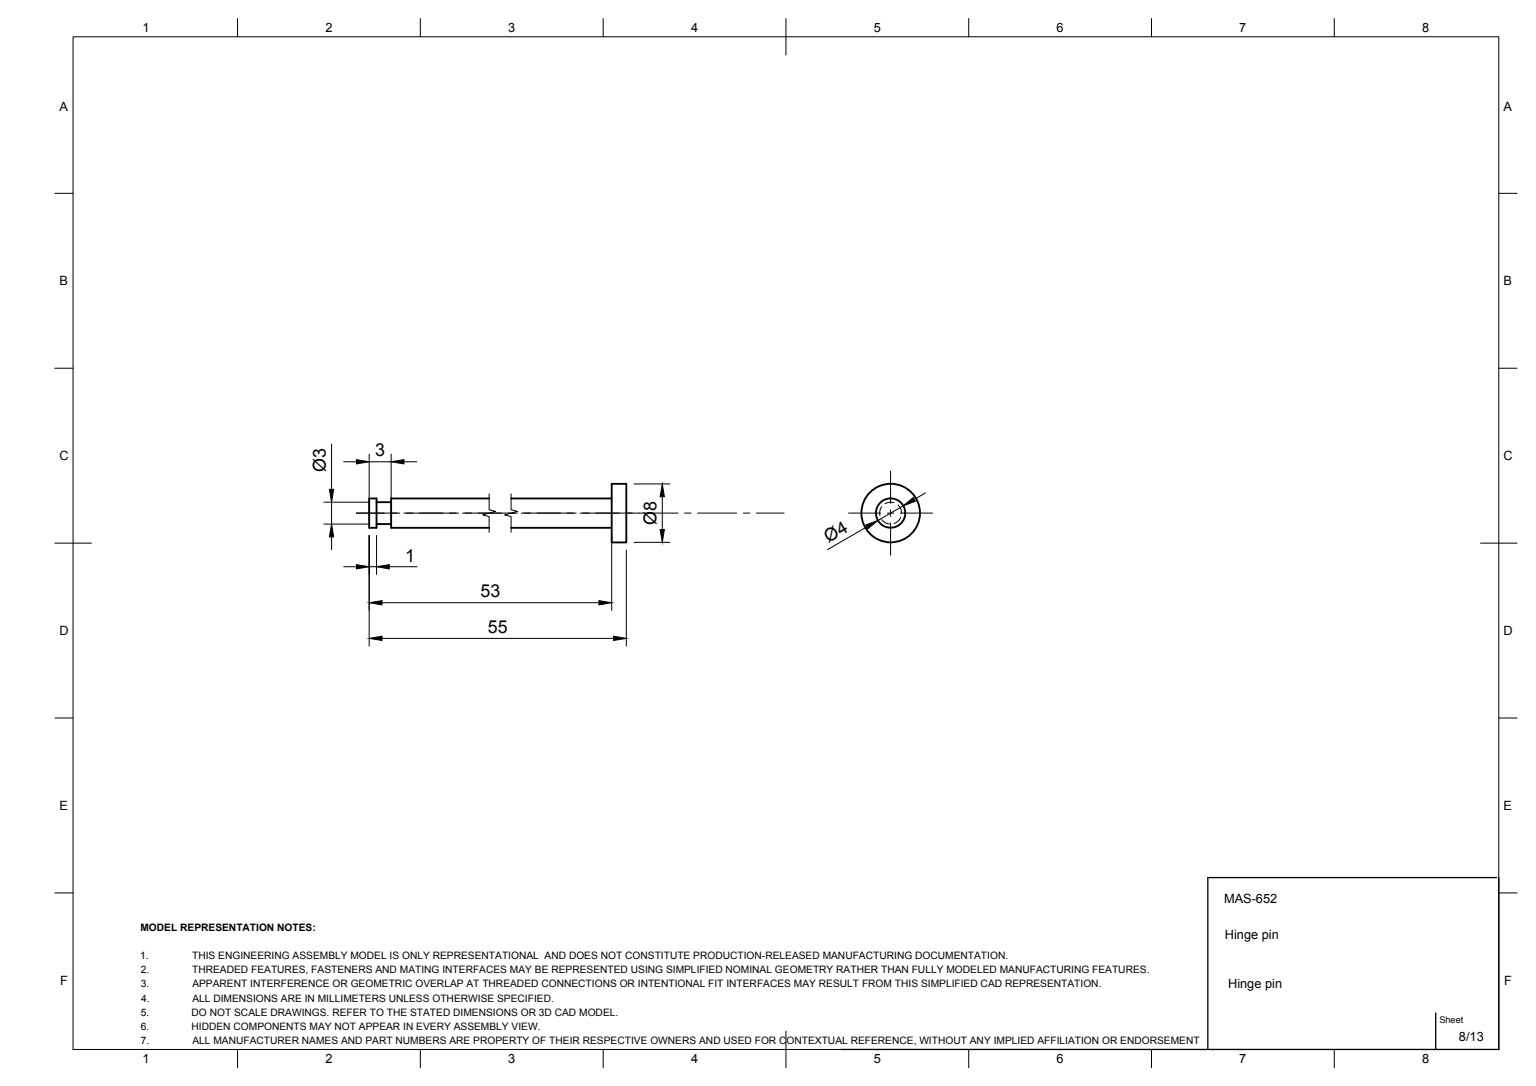
ISO-10303-21;
HEADER;
/* Generated by software containing ST-Developer
 * from STEP Tools, Inc. (www.steptools.com) 
 */

FILE_DESCRIPTION(
/* description */ ('Independent hinged machine back cover with retained hinge pins, perim
eter gasket and quarter-turn cam latch. Nominal cover 360 x 260 x 3 mm
, frame 430 x 300 x 20 mm. No guarding, structural or ingress rating a
ssigned.'),
/* implementation_level */ '2;1');

FILE_NAME(
/* name */ 'Hinge pin.step',
/* time_stamp */ '2026-11-09T19:36:59-08:00',
/* author */ (''),
/* organization */ (''),
/* preprocessor_version */ 'ST-DEVELOPER v20.2',
/* originating_system */ 'Autodesk Translation Framework v15.17.0.0',
/* authorisation */ '');

FILE_SCHEMA (('AUTOMOTIVE_DESIGN { 1 0 10303 214 3 1 1 }'));
ENDSEC;

DATA;
#10=MECHANICAL_DESIGN_GEOMETRIC_PRESENTATION_REPRESENTATION('',(#208),#32627);
#172=SHAPE_REPRESENTATION_RELATIONSHIP('SRR','None',#32718,#190);
#190=ADVANCED_BREP_SHAPE_REPRESENTATION('',(#226),#32619);
#208=STYLED_ITEM('',(#32812),#226);
#226=MANIFOLD_SOLID_BREP('Body1',#8685);
#274=FACE_BOUND('',#1294,.T.);
#275=FACE_BOUND('',#1296,.T.);
#276=FACE_BOUND('',#1299,.T.);
#402=PLANE('',#9298);
#403=PLANE('',#9300);
#404=PLANE('',#9304);
#405=PLANE('',#9309);
#406=PLANE('',#9311);
#777=FACE_OUTER_BOUND('',#1292,.T.);
#778=FACE_OUTER_BOUND('',#1293,.T.);
#779=FACE_OUTER_BOUND('',#1295,.T.);
#780=FACE_OUTER_BOUND('',#1297,.T.);
#781=FACE_OUTER_BOUND('',#1298,.T.);
#782=FACE_OUTER_BOUND('',#1300,.T.);
#783=FACE_OUTER_BOUND('',#1301,.T.);
#784=FACE_OUTER_BOUND('',#1302,.T.);
#785=FACE_OUTER_BOUND('',#1303,.T.);
#1292=EDGE_LOOP('',(#7125,#7126,#7127,#7128));
#1293=EDGE_LOOP('',(#7129));
#1294=EDGE_LOOP('',(#7130));
#1295=EDGE_LOOP('',(#7131));
#1296=EDGE_LOOP('',(#7132));
#1297=EDGE_LOOP('',(#7133,#7134,#7135,#7136));
#1298=EDGE_LOOP('',(#7137));
#1299=EDGE_LOOP('',(#7138));
#1300=EDGE_LOOP('',(#7139,#7140,#7141,#7142));
#1301=EDGE_LOOP('',(#7143));
#1302=EDGE_LOOP('',(#7144,#7145,#7146,#7147));
#1303=EDGE_LOOP('',(#7148));
#1539=CIRCLE('',#9296,1.5);
#1540=CIRCLE('',#9297,1.5);
#1541=CIRCLE('',#9299,2.);
#1542=CIRCLE('',#9301,2.);
#1543=CIRCLE('',#9303,2.);
#1544=CIRCLE('',#9305,4.);
#1545=CIRCLE('',#9306,2.);
#1546=CIRCLE('',#9308,4.);
#2552=LINE('',#26260,#3098);
#2553=LINE('',#26271,#3099);
#2554=LINE('',#26279,#3100);
#2555=LINE('',#26283,#3101);
#3098=VECTOR('',#10716,1.5);
#3099=VECTOR('',#10731,2.);
#3100=VECTOR('',#10740,4.);
#3101=VECTOR('',#10747,2.);
#3853=VERTEX_POINT('',#26257);
#3854=VERTEX_POINT('',#26259);
#3855=VERTEX_POINT('',#26263);
#3856=VERTEX_POINT('',#26266);
#3857=VERTEX_POINT('',#26269);
#3858=VERTEX_POINT('',#26273);
#3859=VERTEX_POINT('',#26275);
#3860=VERTEX_POINT('',#26278);
#4986=EDGE_CURVE('',#3853,#3853,#1539,.T.);
#4987=EDGE_CURVE('',#3853,#3854,#2552,.T.);
#4988=EDGE_CURVE('',#3854,#3854,#1540,.T.);
#4989=EDGE_CURVE('',#3855,#3855,#1541,.T.);
#4990=EDGE_CURVE('',#3856,#3856,#1542,.T.);
#4991=EDGE_CURVE('',#3857,#3857,#1543,.T.);
#4992=EDGE_CURVE('',#3857,#3856,#2553,.T.);
#4993=EDGE_CURVE('',#3858,#3858,#1544,.T.);
#4994=EDGE_CURVE('',#3859,#3859,#1545,.T.);
#4995=EDGE_CURVE('',#3858,#3860,#2554,.T.);
#4996=EDGE_CURVE('',#3860,#3860,#1546,.T.);
#4997=EDGE_CURVE('',#3855,#3859,#2555,.T.);
#7125=ORIENTED_EDGE('',*,*,#4986,.T.);
#7126=ORIENTED_EDGE('',*,*,#4987,.T.);
#7127=ORIENTED_EDGE('',*,*,#4988,.F.);
#7128=ORIENTED_EDGE('',*,*,#4987,.F.);
#7129=ORIENTED_EDGE('',*,*,#4989,.F.);
#7130=ORIENTED_EDGE('',*,*,#4986,.F.);
#7131=ORIENTED_EDGE('',*,*,#4990,.F.);
#7132=ORIENTED_EDGE('',*,*,#4988,.T.);
#7133=ORIENTED_EDGE('',*,*,#4991,.F.);
#7134=ORIENTED_EDGE('',*,*,#4992,.T.);
#7135=ORIENTED_EDGE('',*,*,#4990,.T.);
#7136=ORIENTED_EDGE('',*,*,#4992,.F.);
#7137=ORIENTED_EDGE('',*,*,#4993,.T.);
#7138=ORIENTED_EDGE('',*,*,#4994,.F.);
#7139=ORIENTED_EDGE('',*,*,#4993,.F.);
#7140=ORIENTED_EDGE('',*,*,#4995,.T.);
#7141=ORIENTED_EDGE('',*,*,#4996,.T.);
#7142=ORIENTED_EDGE('',*,*,#4995,.F.);
#7143=ORIENTED_EDGE('',*,*,#4996,.F.);
#7144=ORIENTED_EDGE('',*,*,#4989,.T.);
#7145=ORIENTED_EDGE('',*,*,#4997,.T.);
#7146=ORIENTED_EDGE('',*,*,#4994,.T.);
#7147=ORIENTED_EDGE('',*,*,#4997,.F.);
#7148=ORIENTED_EDGE('',*,*,#4991,.T.);
#8108=CYLINDRICAL_SURFACE('',#9295,1.5);
#8109=CYLINDRICAL_SURFACE('',#9302,2.);
#8110=CYLINDRICAL_SURFACE('',#9307,4.);
#8111=CYLINDRICAL_SURFACE('',#9310,2.);
#8525=ADVANCED_FACE('',(#777),#8108,.T.);
#8526=ADVANCED_FACE('',(#778,#274),#402,.F.);
#8527=ADVANCED_FACE('',(#779,#275),#403,.F.);
#8528=ADVANCED_FACE('',(#780),#8109,.T.);
#8529=ADVANCED_FACE('',(#781,#276),#404,.T.);
#8530=ADVANCED_FACE('',(#782),#8110,.T.);
#8531=ADVANCED_FACE('',(#783),#405,.F.);
#8532=ADVANCED_FACE('',(#784),#8111,.T.);
#8533=ADVANCED_FACE('',(#785),#406,.T.);
#8685=CLOSED_SHELL('',(#8525,#8526,#8527,#8528,#8529,#8530,#8531,#8532,
#8533));
#9294=AXIS2_PLACEMENT_3D('',#26255,#10710,#10711);
#9295=AXIS2_PLACEMENT_3D('',#26256,#10712,#10713);
#9296=AXIS2_PLACEMENT_3D('',#26258,#10714,#10715);
#9297=AXIS2_PLACEMENT_3D('',#26261,#10717,#10718);
#9298=AXIS2_PLACEMENT_3D('',#26262,#10719,#10720);
#9299=AXIS2_PLACEMENT_3D('',#26264,#10721,#10722);
#9300=AXIS2_PLACEMENT_3D('',#26265,#10723,#10724);
#9301=AXIS2_PLACEMENT_3D('',#26267,#10725,#10726);
#9302=AXIS2_PLACEMENT_3D('',#26268,#10727,#10728);
#9303=AXIS2_PLACEMENT_3D('',#26270,#10729,#10730);
#9304=AXIS2_PLACEMENT_3D('',#26272,#10732,#10733);
#9305=AXIS2_PLACEMENT_3D('',#26274,#10734,#10735);
#9306=AXIS2_PLACEMENT_3D('',#26276,#10736,#10737);
#9307=AXIS2_PLACEMENT_3D('',#26277,#10738,#10739);
#9308=AXIS2_PLACEMENT_3D('',#26280,#10741,#10742);
#9309=AXIS2_PLACEMENT_3D('',#26281,#10743,#10744);
#9310=AXIS2_PLACEMENT_3D('',#26282,#10745,#10746);
#9311=AXIS2_PLACEMENT_3D('',#26284,#10748,#10749);
#10710=DIRECTION('axis',(0.,0.,1.));
#10711=DIRECTION('refdir',(1.,0.,0.));
#10712=DIRECTION('center_axis',(0.,0.,1.));
#10713=DIRECTION('ref_axis',(1.,0.,0.));
#10714=DIRECTION('center_axis',(0.,0.,1.));
#10715=DIRECTION('ref_axis',(1.,0.,0.));
#10716=DIRECTION('',(0.,0.,1.));
#10717=DIRECTION('center_axis',(0.,0.,1.));
#10718=DIRECTION('ref_axis',(1.,0.,0.));
#10719=DIRECTION('center_axis',(0.,0.,-1.));
#10720=DIRECTION('ref_axis',(-1.,0.,0.));
#10721=DIRECTION('center_axis',(0.,0.,-1.));
#10722=DIRECTION('ref_axis',(1.,0.,0.));
#10723=DIRECTION('center_axis',(0.,0.,1.));
#10724=DIRECTION('ref_axis',(1.,0.,0.));
#10725=DIRECTION('center_axis',(0.,0.,1.));
#10726=DIRECTION('ref_axis',(1.,0.,0.));
#10727=DIRECTION('center_axis',(0.,0.,1.));
#10728=DIRECTION('ref_axis',(1.,0.,0.));
#10729=DIRECTION('center_axis',(0.,0.,1.));
#10730=DIRECTION('ref_axis',(1.,0.,0.));
#10731=DIRECTION('',(0.,0.,-1.));
#10732=DIRECTION('center_axis',(0.,0.,1.));
#10733=DIRECTION('ref_axis',(1.,0.,0.));
#10734=DIRECTION('center_axis',(0.,0.,1.));
#10735=DIRECTION('ref_axis',(1.,0.,0.));
#10736=DIRECTION('center_axis',(0.,0.,1.));
#10737=DIRECTION('ref_axis',(1.,0.,0.));
#10738=DIRECTION('center_axis',(0.,0.,1.));
#10739=DIRECTION('ref_axis',(1.,0.,0.));
#10740=DIRECTION('',(0.,0.,-1.));
#10741=DIRECTION('center_axis',(0.,0.,1.));
#10742=DIRECTION('ref_axis',(1.,0.,0.));
#10743=DIRECTION('center_axis',(0.,0.,1.));
#10744=DIRECTION('ref_axis',(1.,0.,0.));
#10745=DIRECTION('center_axis',(0.,0.,1.));
#10746=DIRECTION('ref_axis',(1.,0.,0.));
#10747=DIRECTION('',(0.,0.,-1.));
#10748=DIRECTION('center_axis',(0.,0.,1.));
#10749=DIRECTION('ref_axis',(1.,0.,0.));
#26255=CARTESIAN_POINT('',(0.,0.,0.));
#26256=CARTESIAN_POINT('Origin',(0.,0.,51.));
#26257=CARTESIAN_POINT('',(-1.5,-1.83697019872103E-16,50.));
#26258=CARTESIAN_POINT('Origin',(0.,0.,50.));
#26259=CARTESIAN_POINT('',(-1.5,-1.83697019872103E-16,52.));
#26260=CARTESIAN_POINT('',(-1.5,-1.83697019872103E-16,51.));
#26261=CARTESIAN_POINT('Origin',(0.,0.,52.));
#26262=CARTESIAN_POINT('Origin',(5.5,0.,50.));
#26263=CARTESIAN_POINT('',(-2.,2.44929359829471E-16,50.));
#26264=CARTESIAN_POINT('Origin',(0.,0.,50.));
#26265=CARTESIAN_POINT('Origin',(1.5,0.,52.));
#26266=CARTESIAN_POINT('',(-2.,-2.44929359829471E-16,52.));
#26267=CARTESIAN_POINT('Origin',(0.,0.,52.));
#26268=CARTESIAN_POINT('Origin',(0.,0.,0.));
#26269=CARTESIAN_POINT('',(-2.,-2.44929359829471E-16,53.));
#26270=CARTESIAN_POINT('Origin',(0.,0.,53.));
#26271=CARTESIAN_POINT('',(-2.,-2.44929359829471E-16,0.));
#26272=CARTESIAN_POINT('Origin',(0.,0.,0.));
#26273=CARTESIAN_POINT('',(-4.,-4.89858719658941E-16,0.));
#26274=CARTESIAN_POINT('Origin',(0.,0.,0.));
#26275=CARTESIAN_POINT('',(-2.,-2.44929359829471E-16,0.));
#26276=CARTESIAN_POINT('Origin',(0.,0.,0.));
#26277=CARTESIAN_POINT('Origin',(0.,0.,-2.));
#26278=CARTESIAN_POINT('',(-4.,-4.89858719658941E-16,-2.));
#26279=CARTESIAN_POINT('',(-4.,-4.89858719658941E-16,-2.));
#26280=CARTESIAN_POINT('Origin',(0.,0.,-2.));
#26281=CARTESIAN_POINT('Origin',(0.,0.,-2.));
#26282=CARTESIAN_POINT('Origin',(0.,0.,0.));
#26283=CARTESIAN_POINT('',(-2.,-2.44929359829471E-16,0.));
#26284=CARTESIAN_POINT('Origin',(0.,0.,53.));
#32599=UNCERTAINTY_MEASURE_WITH_UNIT(LENGTH_MEASURE(0.01),#32628,
'DISTANCE_ACCURACY_VALUE',
'Maximum model space distance between geometric entities at asserted c
onnectivities');
#32607=UNCERTAINTY_MEASURE_WITH_UNIT(LENGTH_MEASURE(0.01),#32628,
'DISTANCE_ACCURACY_VALUE',
'Maximum model space distance between geometric entities at asserted c
onnectivities');
#32619=(
GEOMETRIC_REPRESENTATION_CONTEXT(3)
GLOBAL_UNCERTAINTY_ASSIGNED_CONTEXT((#32599))
GLOBAL_UNIT_ASSIGNED_CONTEXT((#32628,#32630,#32631))
REPRESENTATION_CONTEXT('','3D')
);
#32627=(
GEOMETRIC_REPRESENTATION_CONTEXT(3)
GLOBAL_UNCERTAINTY_ASSIGNED_CONTEXT((#32607))
GLOBAL_UNIT_ASSIGNED_CONTEXT((#32628,#32630,#32631))
REPRESENTATION_CONTEXT('','3D')
);
#32628=(
LENGTH_UNIT()
NAMED_UNIT(*)
SI_UNIT(.MILLI.,.METRE.)
);
#32630=(
NAMED_UNIT(*)
PLANE_ANGLE_UNIT()
SI_UNIT($,.RADIAN.)
);
#32631=(
NAMED_UNIT(*)
SI_UNIT($,.STERADIAN.)
SOLID_ANGLE_UNIT()
);
#32643=SHAPE_DEFINITION_REPRESENTATION(#32662,#32718);
#32662=PRODUCT_DEFINITION_SHAPE('',$,#32738);
#32718=SHAPE_REPRESENTATION('',(#9294),#32619);
#32726=PRODUCT_DEFINITION_CONTEXT('part definition',#32785,'design');
#32738=PRODUCT_DEFINITION('Hinge pin','Hinge pin',#32757,#32726);
#32757=PRODUCT_DEFINITION_FORMATION('',$,#32798);
#32785=APPLICATION_CONTEXT(
'Core Data for Automotive Mechanical Design Process');
#32786=PRODUCT_CONTEXT('part definition',#32785,'mechanical');
#32798=PRODUCT('Hinge pin','Hinge pin','Hinge pin',(#32786));
#32812=PRESENTATION_STYLE_ASSIGNMENT((#32819));
#32819=SURFACE_STYLE_USAGE(.BOTH.,#32826);
#32826=SURFACE_SIDE_STYLE('',(#32833));
#32833=SURFACE_STYLE_FILL_AREA(#32840);
#32840=FILL_AREA_STYLE('Light gray',(#32847));
#32847=FILL_AREA_STYLE_COLOUR('Light gray',#32854);
#32854=COLOUR_RGB('Light gray',0.725490196078431,0.752941176470588,0.792156862745098);
ENDSEC;
END-ISO-10303-21;
